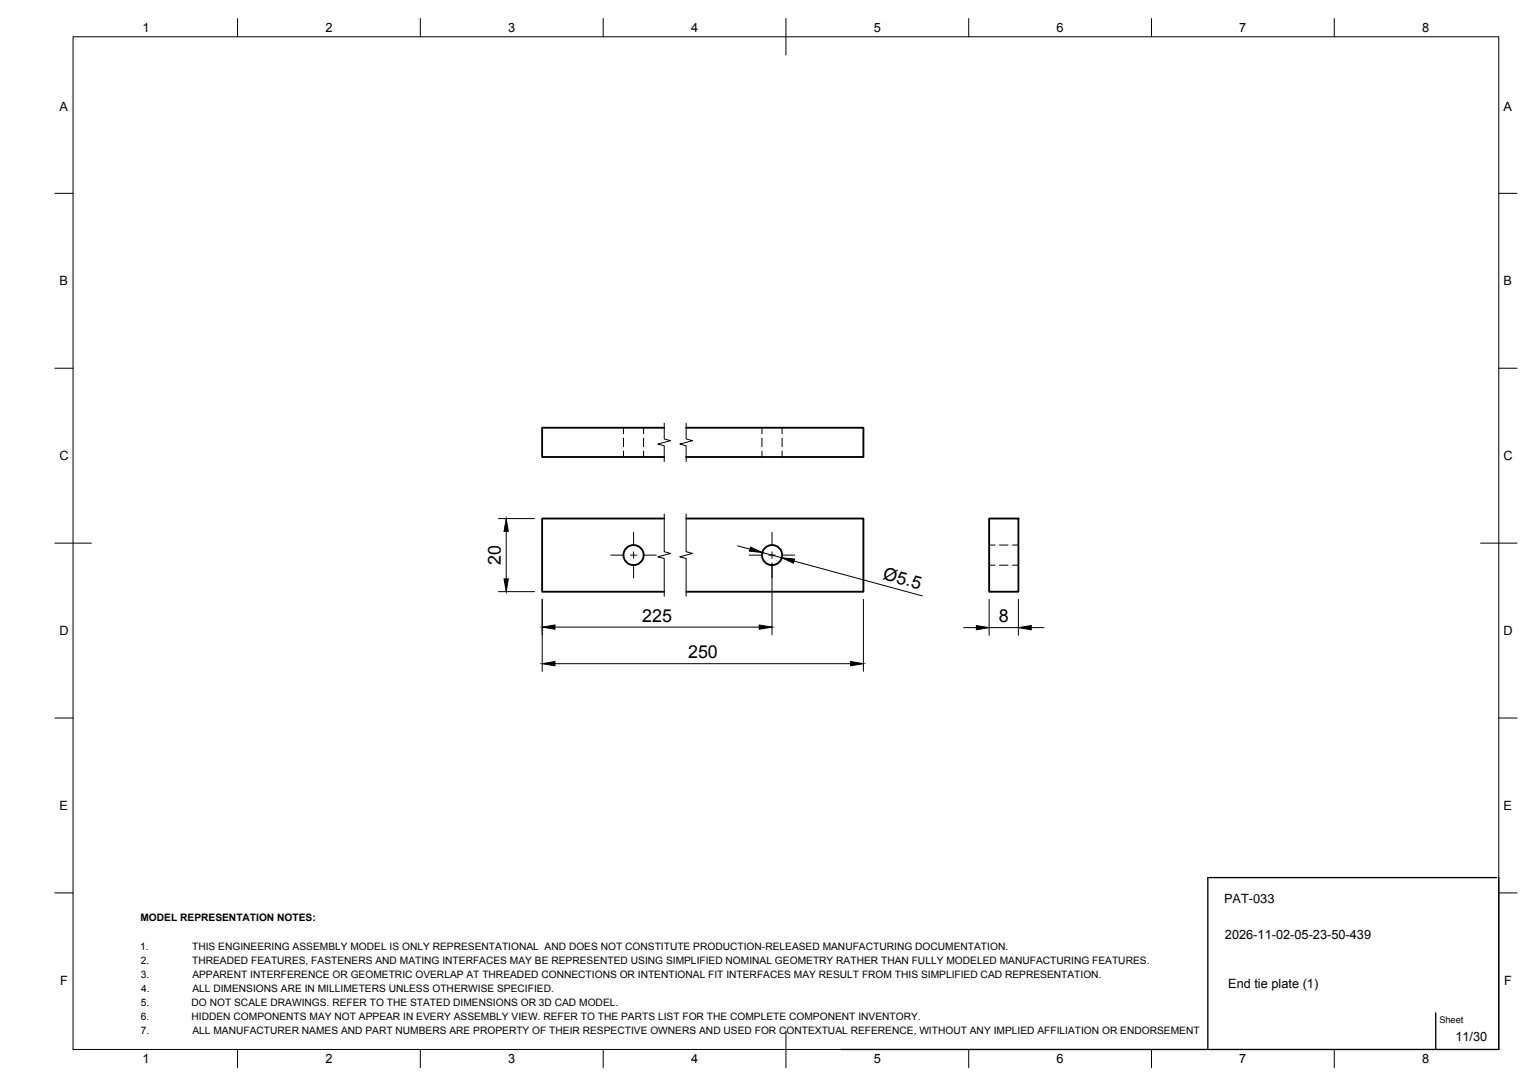
ISO-10303-21;
HEADER;
/* Generated by software containing ST-Developer
 * from STEP Tools, Inc. (www.steptools.com) 
 */

FILE_DESCRIPTION(
/* description */ ('Dual-rail gantry carriage'),
/* implementation_level */ '2;1');

FILE_NAME(
/* name */ 'End tie plate (1).step',
/* time_stamp */ '2026-10-27T10:49:15-07:00',
/* author */ (''),
/* organization */ (''),
/* preprocessor_version */ 'ST-DEVELOPER v20.2',
/* originating_system */ 'Autodesk Translation Framework v15.17.0.0',
/* authorisation */ '');

FILE_SCHEMA (('AUTOMOTIVE_DESIGN { 1 0 10303 214 3 1 1 }'));
ENDSEC;

DATA;
#10=MECHANICAL_DESIGN_GEOMETRIC_PRESENTATION_REPRESENTATION('',(#591),#12804);
#529=SHAPE_REPRESENTATION_RELATIONSHIP('SRR','None',#13007,#560);
#560=ADVANCED_BREP_SHAPE_REPRESENTATION('',(#622),#12777);
#591=STYLED_ITEM('',(#13233),#622);
#622=MANIFOLD_SOLID_BREP('Body1',#7369);
#674=FACE_BOUND('',#1528,.T.);
#675=FACE_BOUND('',#1529,.T.);
#676=FACE_BOUND('',#1531,.T.);
#677=FACE_BOUND('',#1532,.T.);
#800=PLANE('',#7840);
#801=PLANE('',#7841);
#802=PLANE('',#7842);
#803=PLANE('',#7843);
#804=PLANE('',#7844);
#805=PLANE('',#7845);
#1100=FACE_OUTER_BOUND('',#1521,.T.);
#1101=FACE_OUTER_BOUND('',#1522,.T.);
#1102=FACE_OUTER_BOUND('',#1523,.T.);
#1103=FACE_OUTER_BOUND('',#1524,.T.);
#1104=FACE_OUTER_BOUND('',#1525,.T.);
#1105=FACE_OUTER_BOUND('',#1526,.T.);
#1106=FACE_OUTER_BOUND('',#1527,.T.);
#1107=FACE_OUTER_BOUND('',#1530,.T.);
#1521=EDGE_LOOP('',(#5307,#5308,#5309,#5310));
#1522=EDGE_LOOP('',(#5311,#5312,#5313,#5314));
#1523=EDGE_LOOP('',(#5315,#5316,#5317,#5318));
#1524=EDGE_LOOP('',(#5319,#5320,#5321,#5322));
#1525=EDGE_LOOP('',(#5323,#5324,#5325,#5326));
#1526=EDGE_LOOP('',(#5327,#5328,#5329,#5330));
#1527=EDGE_LOOP('',(#5331,#5332,#5333,#5334));
#1528=EDGE_LOOP('',(#5335));
#1529=EDGE_LOOP('',(#5336));
#1530=EDGE_LOOP('',(#5337,#5338,#5339,#5340));
#1531=EDGE_LOOP('',(#5341));
#1532=EDGE_LOOP('',(#5342));
#2036=LINE('',#10953,#2745);
#2037=LINE('',#10959,#2746);
#2038=LINE('',#10964,#2747);
#2039=LINE('',#10966,#2748);
#2040=LINE('',#10968,#2749);
#2041=LINE('',#10969,#2750);
#2042=LINE('',#10972,#2751);
#2043=LINE('',#10974,#2752);
#2044=LINE('',#10975,#2753);
#2045=LINE('',#10978,#2754);
#2046=LINE('',#10980,#2755);
#2047=LINE('',#10981,#2756);
#2048=LINE('',#10983,#2757);
#2049=LINE('',#10984,#2758);
#2745=VECTOR('',#8765,0.274999999999999);
#2746=VECTOR('',#8772,0.274999999999999);
#2747=VECTOR('',#8777,1.);
#2748=VECTOR('',#8778,1.);
#2749=VECTOR('',#8779,1.);
#2750=VECTOR('',#8780,1.);
#2751=VECTOR('',#8783,1.);
#2752=VECTOR('',#8784,1.);
#2753=VECTOR('',#8785,1.);
#2754=VECTOR('',#8788,1.);
#2755=VECTOR('',#8789,1.);
#2756=VECTOR('',#8790,1.);
#2757=VECTOR('',#8793,1.);
#2758=VECTOR('',#8794,1.);
#3398=CIRCLE('',#7835,0.274999999999999);
#3399=CIRCLE('',#7836,0.274999999999999);
#3400=CIRCLE('',#7838,0.274999999999999);
#3401=CIRCLE('',#7839,0.274999999999999);
#3646=VERTEX_POINT('',#10950);
#3647=VERTEX_POINT('',#10952);
#3648=VERTEX_POINT('',#10956);
#3649=VERTEX_POINT('',#10958);
#3650=VERTEX_POINT('',#10962);
#3651=VERTEX_POINT('',#10963);
#3652=VERTEX_POINT('',#10965);
#3653=VERTEX_POINT('',#10967);
#3654=VERTEX_POINT('',#10971);
#3655=VERTEX_POINT('',#10973);
#3656=VERTEX_POINT('',#10977);
#3657=VERTEX_POINT('',#10979);
#4276=EDGE_CURVE('',#3646,#3646,#3398,.T.);
#4277=EDGE_CURVE('',#3646,#3647,#2036,.T.);
#4278=EDGE_CURVE('',#3647,#3647,#3399,.T.);
#4279=EDGE_CURVE('',#3648,#3648,#3400,.T.);
#4280=EDGE_CURVE('',#3648,#3649,#2037,.T.);
#4281=EDGE_CURVE('',#3649,#3649,#3401,.T.);
#4282=EDGE_CURVE('',#3650,#3651,#2038,.T.);
#4283=EDGE_CURVE('',#3651,#3652,#2039,.T.);
#4284=EDGE_CURVE('',#3653,#3652,#2040,.T.);
#4285=EDGE_CURVE('',#3650,#3653,#2041,.T.);
#4286=EDGE_CURVE('',#3654,#3650,#2042,.T.);
#4287=EDGE_CURVE('',#3655,#3653,#2043,.T.);
#4288=EDGE_CURVE('',#3654,#3655,#2044,.T.);
#4289=EDGE_CURVE('',#3656,#3654,#2045,.T.);
#4290=EDGE_CURVE('',#3657,#3655,#2046,.T.);
#4291=EDGE_CURVE('',#3656,#3657,#2047,.T.);
#4292=EDGE_CURVE('',#3651,#3656,#2048,.T.);
#4293=EDGE_CURVE('',#3652,#3657,#2049,.T.);
#5307=ORIENTED_EDGE('',*,*,#4276,.F.);
#5308=ORIENTED_EDGE('',*,*,#4277,.T.);
#5309=ORIENTED_EDGE('',*,*,#4278,.F.);
#5310=ORIENTED_EDGE('',*,*,#4277,.F.);
#5311=ORIENTED_EDGE('',*,*,#4279,.F.);
#5312=ORIENTED_EDGE('',*,*,#4280,.T.);
#5313=ORIENTED_EDGE('',*,*,#4281,.F.);
#5314=ORIENTED_EDGE('',*,*,#4280,.F.);
#5315=ORIENTED_EDGE('',*,*,#4282,.T.);
#5316=ORIENTED_EDGE('',*,*,#4283,.T.);
#5317=ORIENTED_EDGE('',*,*,#4284,.F.);
#5318=ORIENTED_EDGE('',*,*,#4285,.F.);
#5319=ORIENTED_EDGE('',*,*,#4286,.T.);
#5320=ORIENTED_EDGE('',*,*,#4285,.T.);
#5321=ORIENTED_EDGE('',*,*,#4287,.F.);
#5322=ORIENTED_EDGE('',*,*,#4288,.F.);
#5323=ORIENTED_EDGE('',*,*,#4289,.T.);
#5324=ORIENTED_EDGE('',*,*,#4288,.T.);
#5325=ORIENTED_EDGE('',*,*,#4290,.F.);
#5326=ORIENTED_EDGE('',*,*,#4291,.F.);
#5327=ORIENTED_EDGE('',*,*,#4292,.T.);
#5328=ORIENTED_EDGE('',*,*,#4291,.T.);
#5329=ORIENTED_EDGE('',*,*,#4293,.F.);
#5330=ORIENTED_EDGE('',*,*,#4283,.F.);
#5331=ORIENTED_EDGE('',*,*,#4293,.T.);
#5332=ORIENTED_EDGE('',*,*,#4290,.T.);
#5333=ORIENTED_EDGE('',*,*,#4287,.T.);
#5334=ORIENTED_EDGE('',*,*,#4284,.T.);
#5335=ORIENTED_EDGE('',*,*,#4278,.T.);
#5336=ORIENTED_EDGE('',*,*,#4281,.T.);
#5337=ORIENTED_EDGE('',*,*,#4292,.F.);
#5338=ORIENTED_EDGE('',*,*,#4282,.F.);
#5339=ORIENTED_EDGE('',*,*,#4286,.F.);
#5340=ORIENTED_EDGE('',*,*,#4289,.F.);
#5341=ORIENTED_EDGE('',*,*,#4276,.T.);
#5342=ORIENTED_EDGE('',*,*,#4279,.T.);
#6905=CYLINDRICAL_SURFACE('',#7834,0.274999999999999);
#6906=CYLINDRICAL_SURFACE('',#7837,0.274999999999999);
#7026=ADVANCED_FACE('',(#1100),#6905,.F.);
#7027=ADVANCED_FACE('',(#1101),#6906,.F.);
#7028=ADVANCED_FACE('',(#1102),#800,.T.);
#7029=ADVANCED_FACE('',(#1103),#801,.T.);
#7030=ADVANCED_FACE('',(#1104),#802,.T.);
#7031=ADVANCED_FACE('',(#1105),#803,.T.);
#7032=ADVANCED_FACE('',(#1106,#674,#675),#804,.T.);
#7033=ADVANCED_FACE('',(#1107,#676,#677),#805,.F.);
#7369=CLOSED_SHELL('',(#7026,#7027,#7028,#7029,#7030,#7031,#7032,#7033));
#7833=AXIS2_PLACEMENT_3D('',#10948,#8759,#8760);
#7834=AXIS2_PLACEMENT_3D('',#10949,#8761,#8762);
#7835=AXIS2_PLACEMENT_3D('',#10951,#8763,#8764);
#7836=AXIS2_PLACEMENT_3D('',#10954,#8766,#8767);
#7837=AXIS2_PLACEMENT_3D('',#10955,#8768,#8769);
#7838=AXIS2_PLACEMENT_3D('',#10957,#8770,#8771);
#7839=AXIS2_PLACEMENT_3D('',#10960,#8773,#8774);
#7840=AXIS2_PLACEMENT_3D('',#10961,#8775,#8776);
#7841=AXIS2_PLACEMENT_3D('',#10970,#8781,#8782);
#7842=AXIS2_PLACEMENT_3D('',#10976,#8786,#8787);
#7843=AXIS2_PLACEMENT_3D('',#10982,#8791,#8792);
#7844=AXIS2_PLACEMENT_3D('',#10985,#8795,#8796);
#7845=AXIS2_PLACEMENT_3D('',#10986,#8797,#8798);
#8759=DIRECTION('axis',(0.,0.,1.));
#8760=DIRECTION('refdir',(1.,0.,0.));
#8761=DIRECTION('center_axis',(0.,0.,1.));
#8762=DIRECTION('ref_axis',(1.,0.,0.));
#8763=DIRECTION('center_axis',(0.,0.,1.));
#8764=DIRECTION('ref_axis',(1.,0.,0.));
#8765=DIRECTION('',(0.,0.,1.));
#8766=DIRECTION('center_axis',(0.,0.,-1.));
#8767=DIRECTION('ref_axis',(1.,0.,0.));
#8768=DIRECTION('center_axis',(0.,0.,1.));
#8769=DIRECTION('ref_axis',(1.,0.,0.));
#8770=DIRECTION('center_axis',(0.,0.,1.));
#8771=DIRECTION('ref_axis',(1.,0.,0.));
#8772=DIRECTION('',(0.,0.,1.));
#8773=DIRECTION('center_axis',(0.,0.,-1.));
#8774=DIRECTION('ref_axis',(1.,0.,0.));
#8775=DIRECTION('center_axis',(0.,1.,0.));
#8776=DIRECTION('ref_axis',(-1.,0.,0.));
#8777=DIRECTION('',(-1.,0.,0.));
#8778=DIRECTION('',(0.,0.,1.));
#8779=DIRECTION('',(-1.,0.,0.));
#8780=DIRECTION('',(0.,0.,1.));
#8781=DIRECTION('center_axis',(1.,0.,0.));
#8782=DIRECTION('ref_axis',(0.,1.,0.));
#8783=DIRECTION('',(0.,1.,0.));
#8784=DIRECTION('',(0.,1.,0.));
#8785=DIRECTION('',(0.,0.,1.));
#8786=DIRECTION('center_axis',(0.,-1.,0.));
#8787=DIRECTION('ref_axis',(1.,0.,0.));
#8788=DIRECTION('',(1.,0.,0.));
#8789=DIRECTION('',(1.,0.,0.));
#8790=DIRECTION('',(0.,0.,1.));
#8791=DIRECTION('center_axis',(-1.,0.,0.));
#8792=DIRECTION('ref_axis',(0.,-1.,0.));
#8793=DIRECTION('',(0.,-1.,0.));
#8794=DIRECTION('',(0.,-1.,0.));
#8795=DIRECTION('center_axis',(0.,0.,1.));
#8796=DIRECTION('ref_axis',(1.,0.,0.));
#8797=DIRECTION('center_axis',(0.,0.,1.));
#8798=DIRECTION('ref_axis',(1.,0.,0.));
#10948=CARTESIAN_POINT('',(0.,0.,0.));
#10949=CARTESIAN_POINT('Origin',(39.,-10.,-0.9));
#10950=CARTESIAN_POINT('',(38.725,-10.,2.));
#10951=CARTESIAN_POINT('Origin',(39.,-10.,2.));
#10952=CARTESIAN_POINT('',(38.725,-10.,2.8));
#10953=CARTESIAN_POINT('',(38.725,-10.,-0.9));
#10954=CARTESIAN_POINT('Origin',(39.,-10.,2.8));
#10955=CARTESIAN_POINT('Origin',(39.,10.,-0.9));
#10956=CARTESIAN_POINT('',(38.725,10.,2.));
#10957=CARTESIAN_POINT('Origin',(39.,10.,2.));
#10958=CARTESIAN_POINT('',(38.725,10.,2.8));
#10959=CARTESIAN_POINT('',(38.725,10.,-0.9));
#10960=CARTESIAN_POINT('Origin',(39.,10.,2.8));
#10961=CARTESIAN_POINT('Origin',(40.,12.5,2.));
#10962=CARTESIAN_POINT('',(40.,12.5,2.));
#10963=CARTESIAN_POINT('',(38.,12.5,2.));
#10964=CARTESIAN_POINT('',(40.,12.5,2.));
#10965=CARTESIAN_POINT('',(38.,12.5,2.8));
#10966=CARTESIAN_POINT('',(38.,12.5,2.));
#10967=CARTESIAN_POINT('',(40.,12.5,2.8));
#10968=CARTESIAN_POINT('',(40.,12.5,2.8));
#10969=CARTESIAN_POINT('',(40.,12.5,2.));
#10970=CARTESIAN_POINT('Origin',(40.,-12.5,2.));
#10971=CARTESIAN_POINT('',(40.,-12.5,2.));
#10972=CARTESIAN_POINT('',(40.,-12.5,2.));
#10973=CARTESIAN_POINT('',(40.,-12.5,2.8));
#10974=CARTESIAN_POINT('',(40.,-12.5,2.8));
#10975=CARTESIAN_POINT('',(40.,-12.5,2.));
#10976=CARTESIAN_POINT('Origin',(38.,-12.5,2.));
#10977=CARTESIAN_POINT('',(38.,-12.5,2.));
#10978=CARTESIAN_POINT('',(38.,-12.5,2.));
#10979=CARTESIAN_POINT('',(38.,-12.5,2.8));
#10980=CARTESIAN_POINT('',(38.,-12.5,2.8));
#10981=CARTESIAN_POINT('',(38.,-12.5,2.));
#10982=CARTESIAN_POINT('Origin',(38.,12.5,2.));
#10983=CARTESIAN_POINT('',(38.,12.5,2.));
#10984=CARTESIAN_POINT('',(38.,12.5,2.8));
#10985=CARTESIAN_POINT('Origin',(39.,0.,2.8));
#10986=CARTESIAN_POINT('Origin',(39.,0.,2.));
#12741=UNCERTAINTY_MEASURE_WITH_UNIT(LENGTH_MEASURE(0.001),#12805,
'DISTANCE_ACCURACY_VALUE',
'Maximum model space distance between geometric entities at asserted c
onnectivities');
#12768=UNCERTAINTY_MEASURE_WITH_UNIT(LENGTH_MEASURE(0.001),#12805,
'DISTANCE_ACCURACY_VALUE',
'Maximum model space distance between geometric entities at asserted c
onnectivities');
#12777=(
GEOMETRIC_REPRESENTATION_CONTEXT(3)
GLOBAL_UNCERTAINTY_ASSIGNED_CONTEXT((#12741))
GLOBAL_UNIT_ASSIGNED_CONTEXT((#12805,#12807,#12808))
REPRESENTATION_CONTEXT('','3D')
);
#12804=(
GEOMETRIC_REPRESENTATION_CONTEXT(3)
GLOBAL_UNCERTAINTY_ASSIGNED_CONTEXT((#12768))
GLOBAL_UNIT_ASSIGNED_CONTEXT((#12805,#12807,#12808))
REPRESENTATION_CONTEXT('','3D')
);
#12805=(
LENGTH_UNIT()
NAMED_UNIT(*)
SI_UNIT(.CENTI.,.METRE.)
);
#12807=(
NAMED_UNIT(*)
PLANE_ANGLE_UNIT()
SI_UNIT($,.RADIAN.)
);
#12808=(
NAMED_UNIT(*)
SI_UNIT($,.STERADIAN.)
SOLID_ANGLE_UNIT()
);
#12817=SHAPE_DEFINITION_REPRESENTATION(#12852,#13007);
#12852=PRODUCT_DEFINITION_SHAPE('',$,#13043);
#13007=SHAPE_REPRESENTATION('',(#7833),#12777);
#13034=PRODUCT_DEFINITION_CONTEXT('part definition',#13141,'design');
#13043=PRODUCT_DEFINITION('End tie plate (1)','End tie plate (1)',#13078,
#13034);
#13078=PRODUCT_DEFINITION_FORMATION('',$,#13151);
#13141=APPLICATION_CONTEXT(
'Core Data for Automotive Mechanical Design Process');
#13142=PRODUCT_CONTEXT('part definition',#13141,'mechanical');
#13151=PRODUCT('End tie plate (1)','End tie plate (1)','End tie plate (1)',(#13142));
#13227=COLOUR_RGB('Light Blue',0.38,0.62,0.78);
#13228=FILL_AREA_STYLE_COLOUR('',#13227);
#13229=FILL_AREA_STYLE('',(#13228));
#13230=SURFACE_STYLE_FILL_AREA(#13229);
#13231=SURFACE_SIDE_STYLE('',(#13230));
#13232=SURFACE_STYLE_USAGE(.BOTH.,#13231);
#13233=PRESENTATION_STYLE_ASSIGNMENT((#13232));
ENDSEC;
END-ISO-10303-21;
